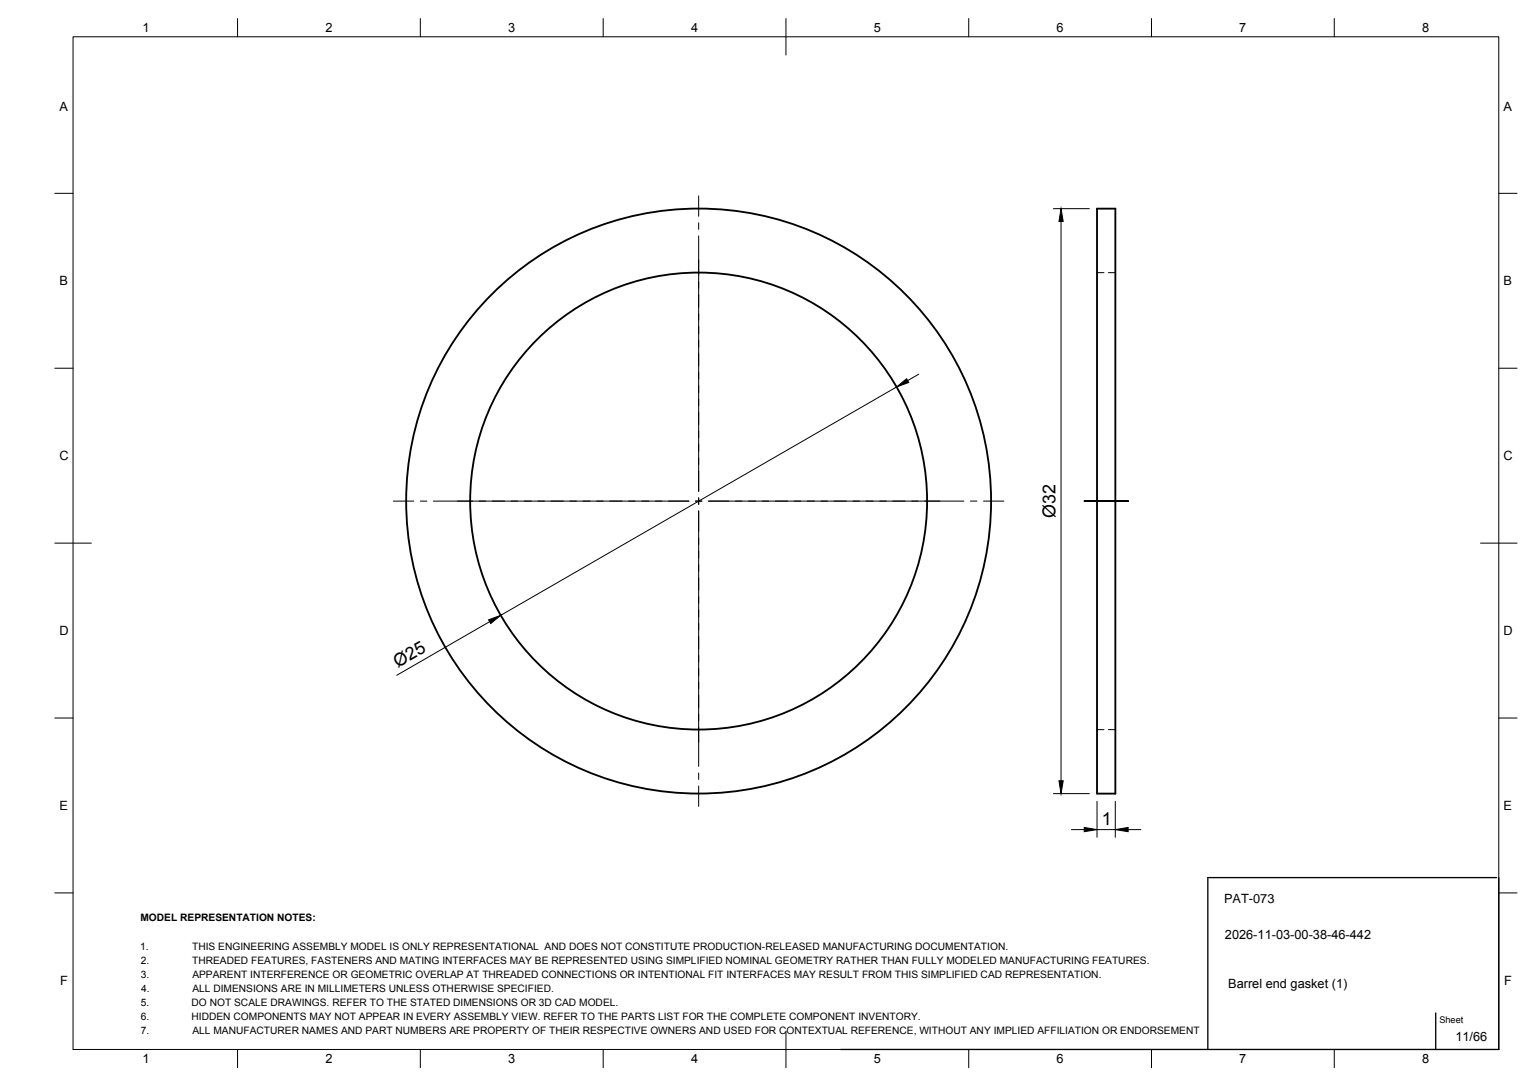
ISO-10303-21;
HEADER;
/* Generated by software containing ST-Developer
 * from STEP Tools, Inc. (www.steptools.com) 
 */

FILE_DESCRIPTION(
/* description */ ('Manual piston pump'),
/* implementation_level */ '2;1');

FILE_NAME(
/* name */ 'Barrel end gasket (1).step',
/* time_stamp */ '2026-11-02T16:54:23-08:00',
/* author */ (''),
/* organization */ (''),
/* preprocessor_version */ 'ST-DEVELOPER v20.2',
/* originating_system */ 'Autodesk Translation Framework v15.17.0.0',
/* authorisation */ '');

FILE_SCHEMA (('AUTOMOTIVE_DESIGN { 1 0 10303 214 3 1 1 }'));
ENDSEC;

DATA;
#10=MECHANICAL_DESIGN_GEOMETRIC_PRESENTATION_REPRESENTATION('',(#694),#19043);
#568=SHAPE_REPRESENTATION_RELATIONSHIP('SRR','None',#19314,#631);
#631=ADVANCED_BREP_SHAPE_REPRESENTATION('',(#766),#18981);
#694=STYLED_ITEM('',(#19661),#766);
#766=MANIFOLD_SOLID_BREP('Body1',#9478);
#878=FACE_BOUND('',#2009,.T.);
#879=FACE_BOUND('',#2011,.T.);
#1132=CYLINDRICAL_SURFACE('',#10424,1.25);
#1133=CYLINDRICAL_SURFACE('',#10427,1.6);
#1380=FACE_OUTER_BOUND('',#2006,.T.);
#1381=FACE_OUTER_BOUND('',#2007,.T.);
#1382=FACE_OUTER_BOUND('',#2008,.T.);
#1383=FACE_OUTER_BOUND('',#2010,.T.);
#2006=EDGE_LOOP('',(#6671,#6672,#6673,#6674));
#2007=EDGE_LOOP('',(#6675,#6676,#6677,#6678));
#2008=EDGE_LOOP('',(#6679));
#2009=EDGE_LOOP('',(#6680));
#2010=EDGE_LOOP('',(#6681));
#2011=EDGE_LOOP('',(#6682));
#2747=CIRCLE('',#10425,1.25);
#2748=CIRCLE('',#10426,1.25);
#2749=CIRCLE('',#10428,1.6);
#2750=CIRCLE('',#10429,1.6);
#3259=LINE('',#15086,#3863);
#3260=LINE('',#15092,#3864);
#3863=VECTOR('',#11973,1.25);
#3864=VECTOR('',#11980,1.6);
#4487=VERTEX_POINT('',#15083);
#4488=VERTEX_POINT('',#15085);
#4489=VERTEX_POINT('',#15089);
#4490=VERTEX_POINT('',#15091);
#5322=EDGE_CURVE('',#4487,#4487,#2747,.T.);
#5323=EDGE_CURVE('',#4487,#4488,#3259,.T.);
#5324=EDGE_CURVE('',#4488,#4488,#2748,.T.);
#5325=EDGE_CURVE('',#4489,#4489,#2749,.T.);
#5326=EDGE_CURVE('',#4489,#4490,#3260,.T.);
#5327=EDGE_CURVE('',#4490,#4490,#2750,.T.);
#6671=ORIENTED_EDGE('',*,*,#5322,.F.);
#6672=ORIENTED_EDGE('',*,*,#5323,.T.);
#6673=ORIENTED_EDGE('',*,*,#5324,.T.);
#6674=ORIENTED_EDGE('',*,*,#5323,.F.);
#6675=ORIENTED_EDGE('',*,*,#5325,.F.);
#6676=ORIENTED_EDGE('',*,*,#5326,.T.);
#6677=ORIENTED_EDGE('',*,*,#5327,.T.);
#6678=ORIENTED_EDGE('',*,*,#5326,.F.);
#6679=ORIENTED_EDGE('',*,*,#5325,.T.);
#6680=ORIENTED_EDGE('',*,*,#5322,.T.);
#6681=ORIENTED_EDGE('',*,*,#5327,.F.);
#6682=ORIENTED_EDGE('',*,*,#5324,.F.);
#8620=PLANE('',#10430);
#8621=PLANE('',#10431);
#8985=ADVANCED_FACE('',(#1380),#1132,.F.);
#8986=ADVANCED_FACE('',(#1381),#1133,.T.);
#8987=ADVANCED_FACE('',(#1382,#878),#8620,.T.);
#8988=ADVANCED_FACE('',(#1383,#879),#8621,.F.);
#9478=CLOSED_SHELL('',(#8985,#8986,#8987,#8988));
#10423=AXIS2_PLACEMENT_3D('',#15081,#11967,#11968);
#10424=AXIS2_PLACEMENT_3D('',#15082,#11969,#11970);
#10425=AXIS2_PLACEMENT_3D('',#15084,#11971,#11972);
#10426=AXIS2_PLACEMENT_3D('',#15087,#11974,#11975);
#10427=AXIS2_PLACEMENT_3D('',#15088,#11976,#11977);
#10428=AXIS2_PLACEMENT_3D('',#15090,#11978,#11979);
#10429=AXIS2_PLACEMENT_3D('',#15093,#11981,#11982);
#10430=AXIS2_PLACEMENT_3D('',#15094,#11983,#11984);
#10431=AXIS2_PLACEMENT_3D('',#15095,#11985,#11986);
#11967=DIRECTION('axis',(0.,0.,1.));
#11968=DIRECTION('refdir',(1.,0.,0.));
#11969=DIRECTION('center_axis',(0.,1.,0.));
#11970=DIRECTION('ref_axis',(1.,0.,0.));
#11971=DIRECTION('center_axis',(0.,-1.,0.));
#11972=DIRECTION('ref_axis',(1.,0.,0.));
#11973=DIRECTION('',(0.,-1.,0.));
#11974=DIRECTION('center_axis',(0.,-1.,0.));
#11975=DIRECTION('ref_axis',(1.,0.,0.));
#11976=DIRECTION('center_axis',(0.,1.,0.));
#11977=DIRECTION('ref_axis',(1.,0.,0.));
#11978=DIRECTION('center_axis',(0.,1.,0.));
#11979=DIRECTION('ref_axis',(1.,0.,0.));
#11980=DIRECTION('',(0.,-1.,0.));
#11981=DIRECTION('center_axis',(0.,1.,0.));
#11982=DIRECTION('ref_axis',(1.,0.,0.));
#11983=DIRECTION('center_axis',(0.,1.,0.));
#11984=DIRECTION('ref_axis',(1.,0.,0.));
#11985=DIRECTION('center_axis',(0.,1.,0.));
#11986=DIRECTION('ref_axis',(1.,0.,0.));
#15081=CARTESIAN_POINT('',(0.,0.,0.));
#15082=CARTESIAN_POINT('Origin',(0.,10.8,4.5));
#15083=CARTESIAN_POINT('',(-1.25,10.9,4.5));
#15084=CARTESIAN_POINT('Origin',(0.,10.9,4.5));
#15085=CARTESIAN_POINT('',(-1.25,10.8,4.5));
#15086=CARTESIAN_POINT('',(-1.25,10.8,4.5));
#15087=CARTESIAN_POINT('Origin',(0.,10.8,4.5));
#15088=CARTESIAN_POINT('Origin',(0.,10.8,4.5));
#15089=CARTESIAN_POINT('',(-1.6,10.9,4.5));
#15090=CARTESIAN_POINT('Origin',(0.,10.9,4.5));
#15091=CARTESIAN_POINT('',(-1.6,10.8,4.5));
#15092=CARTESIAN_POINT('',(-1.6,10.8,4.5));
#15093=CARTESIAN_POINT('Origin',(0.,10.8,4.5));
#15094=CARTESIAN_POINT('Origin',(0.,10.9,4.5));
#15095=CARTESIAN_POINT('Origin',(0.,10.8,4.5));
#18910=UNCERTAINTY_MEASURE_WITH_UNIT(LENGTH_MEASURE(0.001),#19044,
'DISTANCE_ACCURACY_VALUE',
'Maximum model space distance between geometric entities at asserted c
onnectivities');
#18972=UNCERTAINTY_MEASURE_WITH_UNIT(LENGTH_MEASURE(0.001),#19044,
'DISTANCE_ACCURACY_VALUE',
'Maximum model space distance between geometric entities at asserted c
onnectivities');
#18981=(
GEOMETRIC_REPRESENTATION_CONTEXT(3)
GLOBAL_UNCERTAINTY_ASSIGNED_CONTEXT((#18910))
GLOBAL_UNIT_ASSIGNED_CONTEXT((#19044,#19046,#19047))
REPRESENTATION_CONTEXT('','3D')
);
#19043=(
GEOMETRIC_REPRESENTATION_CONTEXT(3)
GLOBAL_UNCERTAINTY_ASSIGNED_CONTEXT((#18972))
GLOBAL_UNIT_ASSIGNED_CONTEXT((#19044,#19046,#19047))
REPRESENTATION_CONTEXT('','3D')
);
#19044=(
LENGTH_UNIT()
NAMED_UNIT(*)
SI_UNIT(.CENTI.,.METRE.)
);
#19046=(
NAMED_UNIT(*)
PLANE_ANGLE_UNIT()
SI_UNIT($,.RADIAN.)
);
#19047=(
NAMED_UNIT(*)
SI_UNIT($,.STERADIAN.)
SOLID_ANGLE_UNIT()
);
#19056=SHAPE_DEFINITION_REPRESENTATION(#19126,#19314);
#19126=PRODUCT_DEFINITION_SHAPE('',$,#19385);
#19314=SHAPE_REPRESENTATION('',(#10423),#18981);
#19376=PRODUCT_DEFINITION_CONTEXT('part definition',#19588,'design');
#19385=PRODUCT_DEFINITION('2026-11-03-00-38-46-442',
'Barrel end gasket (1)',#19455,#19376);
#19455=PRODUCT_DEFINITION_FORMATION('',$,#19598);
#19588=APPLICATION_CONTEXT(
'Core Data for Automotive Mechanical Design Process');
#19589=PRODUCT_CONTEXT('part definition',#19588,'mechanical');
#19598=PRODUCT('2026-11-03-00-38-46-442','Barrel end gasket (1)',
'Barrel end gasket',(#19589));
#19661=PRESENTATION_STYLE_ASSIGNMENT((#19667));
#19667=SURFACE_STYLE_USAGE(.BOTH.,#19673);
#19673=SURFACE_SIDE_STYLE('',(#19679));
#19679=SURFACE_STYLE_FILL_AREA(#19685);
#19685=FILL_AREA_STYLE('CAD Library Painted - Engineering blue',(#19691));
#19691=FILL_AREA_STYLE_COLOUR('CAD Library Painted - Engineering blue',
#19697);
#19697=COLOUR_RGB('CAD Library Painted - Engineering blue',0.12156862745098,
0.356862745098039,0.6);
ENDSEC;
END-ISO-10303-21;
